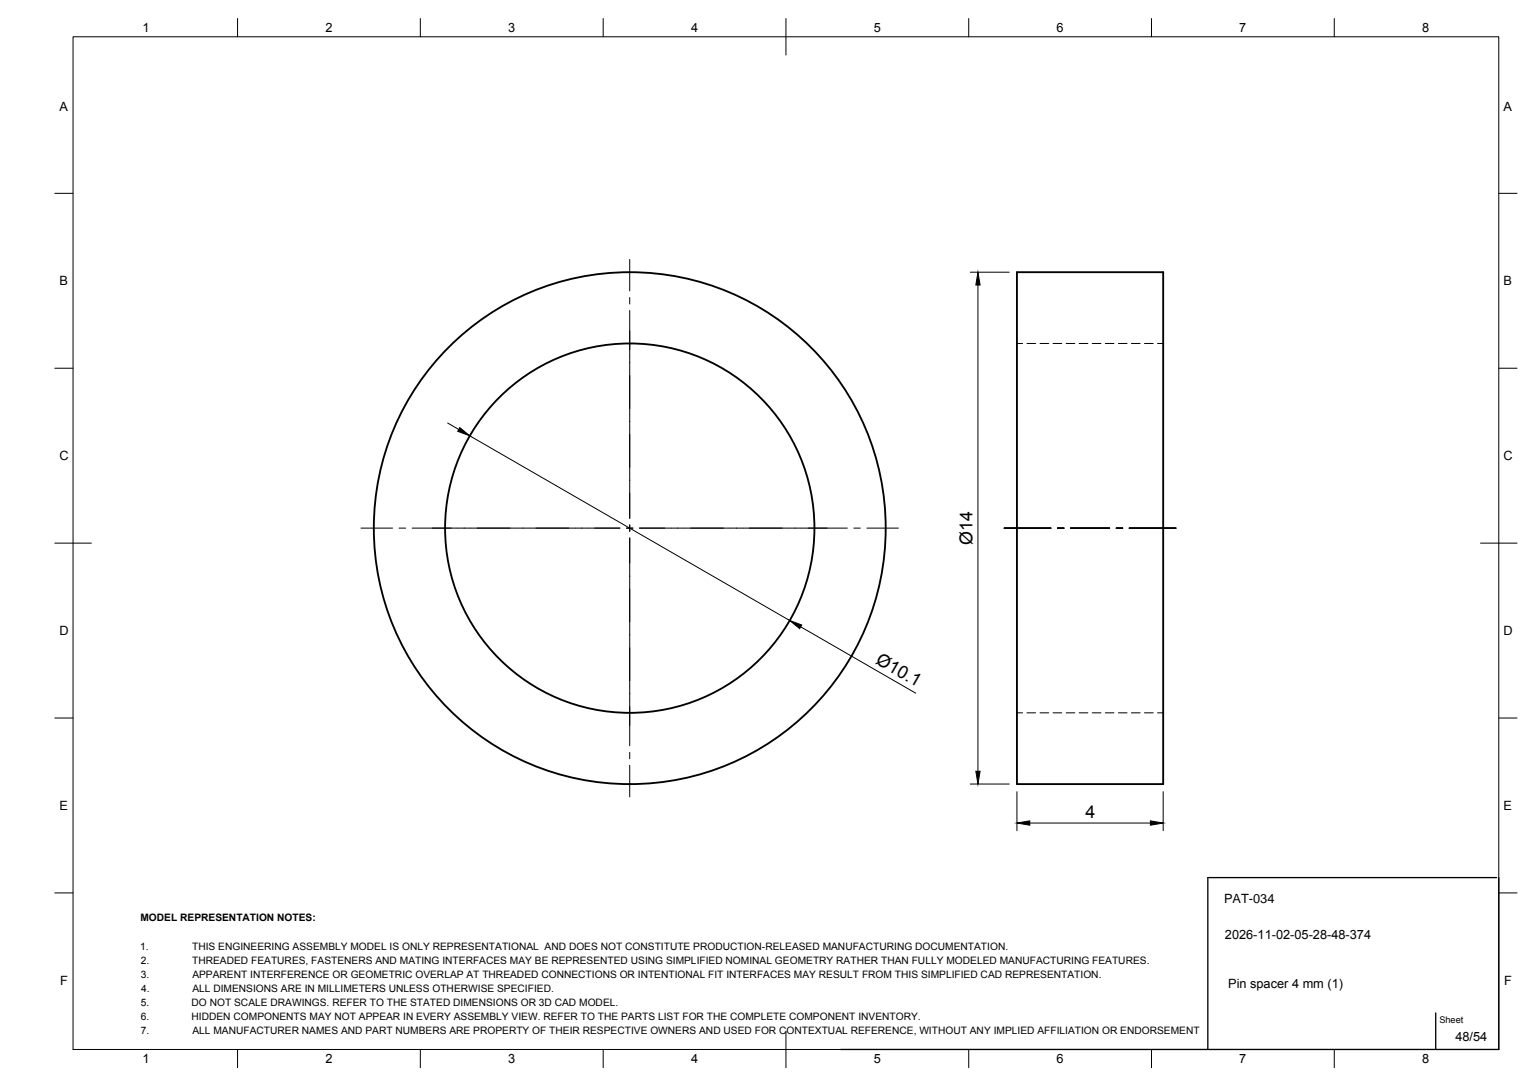
ISO-10303-21;
HEADER;
/* Generated by software containing ST-Developer
 * from STEP Tools, Inc. (www.steptools.com) 
 */

FILE_DESCRIPTION(
/* description */ ('Fatigue rig crank-slider'),
/* implementation_level */ '2;1');

FILE_NAME(
/* name */ 'Pin spacer 4 mm (1).step',
/* time_stamp */ '2026-10-28T03:24:50-07:00',
/* author */ (''),
/* organization */ (''),
/* preprocessor_version */ 'ST-DEVELOPER v20.2',
/* originating_system */ 'Autodesk Translation Framework v15.17.0.0',
/* authorisation */ '');

FILE_SCHEMA (('AUTOMOTIVE_DESIGN { 1 0 10303 214 3 1 1 }'));
ENDSEC;

DATA;
#10=MECHANICAL_DESIGN_GEOMETRIC_PRESENTATION_REPRESENTATION('',(#637),#16911);
#528=SHAPE_REPRESENTATION_RELATIONSHIP('SRR','None',#17172,#578);
#578=ADVANCED_BREP_SHAPE_REPRESENTATION('',(#694),#16901);
#637=STYLED_ITEM('',(#17487),#694);
#694=MANIFOLD_SOLID_BREP('Body1',#8930);
#884=FACE_BOUND('',#2346,.T.);
#885=FACE_BOUND('',#2348,.T.);
#1140=PLANE('',#10330);
#1141=PLANE('',#10331);
#1636=FACE_OUTER_BOUND('',#2343,.T.);
#1637=FACE_OUTER_BOUND('',#2344,.T.);
#1638=FACE_OUTER_BOUND('',#2345,.T.);
#1639=FACE_OUTER_BOUND('',#2347,.T.);
#2343=EDGE_LOOP('',(#7732,#7733,#7734,#7735));
#2344=EDGE_LOOP('',(#7736,#7737,#7738,#7739));
#2345=EDGE_LOOP('',(#7740));
#2346=EDGE_LOOP('',(#7741));
#2347=EDGE_LOOP('',(#7742));
#2348=EDGE_LOOP('',(#7743));
#2925=LINE('',#16224,#3571);
#2926=LINE('',#16230,#3572);
#3571=VECTOR('',#12697,0.505000000000001);
#3572=VECTOR('',#12704,0.699999999999999);
#4101=CIRCLE('',#10325,0.505000000000001);
#4102=CIRCLE('',#10326,0.505000000000001);
#4103=CIRCLE('',#10328,0.699999999999999);
#4104=CIRCLE('',#10329,0.699999999999999);
#4745=VERTEX_POINT('',#16221);
#4746=VERTEX_POINT('',#16223);
#4747=VERTEX_POINT('',#16227);
#4748=VERTEX_POINT('',#16229);
#5764=EDGE_CURVE('',#4745,#4745,#4101,.T.);
#5765=EDGE_CURVE('',#4745,#4746,#2925,.T.);
#5766=EDGE_CURVE('',#4746,#4746,#4102,.T.);
#5767=EDGE_CURVE('',#4747,#4747,#4103,.T.);
#5768=EDGE_CURVE('',#4747,#4748,#2926,.T.);
#5769=EDGE_CURVE('',#4748,#4748,#4104,.T.);
#7732=ORIENTED_EDGE('',*,*,#5764,.F.);
#7733=ORIENTED_EDGE('',*,*,#5765,.T.);
#7734=ORIENTED_EDGE('',*,*,#5766,.T.);
#7735=ORIENTED_EDGE('',*,*,#5765,.F.);
#7736=ORIENTED_EDGE('',*,*,#5767,.F.);
#7737=ORIENTED_EDGE('',*,*,#5768,.T.);
#7738=ORIENTED_EDGE('',*,*,#5769,.T.);
#7739=ORIENTED_EDGE('',*,*,#5768,.F.);
#7740=ORIENTED_EDGE('',*,*,#5767,.T.);
#7741=ORIENTED_EDGE('',*,*,#5764,.T.);
#7742=ORIENTED_EDGE('',*,*,#5769,.F.);
#7743=ORIENTED_EDGE('',*,*,#5766,.F.);
#8339=CYLINDRICAL_SURFACE('',#10324,0.505000000000001);
#8340=CYLINDRICAL_SURFACE('',#10327,0.699999999999999);
#8774=ADVANCED_FACE('',(#1636),#8339,.F.);
#8775=ADVANCED_FACE('',(#1637),#8340,.T.);
#8776=ADVANCED_FACE('',(#1638,#884),#1140,.T.);
#8777=ADVANCED_FACE('',(#1639,#885),#1141,.F.);
#8930=CLOSED_SHELL('',(#8774,#8775,#8776,#8777));
#10323=AXIS2_PLACEMENT_3D('',#16219,#12691,#12692);
#10324=AXIS2_PLACEMENT_3D('',#16220,#12693,#12694);
#10325=AXIS2_PLACEMENT_3D('',#16222,#12695,#12696);
#10326=AXIS2_PLACEMENT_3D('',#16225,#12698,#12699);
#10327=AXIS2_PLACEMENT_3D('',#16226,#12700,#12701);
#10328=AXIS2_PLACEMENT_3D('',#16228,#12702,#12703);
#10329=AXIS2_PLACEMENT_3D('',#16231,#12705,#12706);
#10330=AXIS2_PLACEMENT_3D('',#16232,#12707,#12708);
#10331=AXIS2_PLACEMENT_3D('',#16233,#12709,#12710);
#12691=DIRECTION('axis',(0.,0.,1.));
#12692=DIRECTION('refdir',(1.,0.,0.));
#12693=DIRECTION('center_axis',(0.,1.,0.));
#12694=DIRECTION('ref_axis',(1.,0.,0.));
#12695=DIRECTION('center_axis',(0.,-1.,0.));
#12696=DIRECTION('ref_axis',(1.,0.,0.));
#12697=DIRECTION('',(0.,-1.,0.));
#12698=DIRECTION('center_axis',(0.,-1.,0.));
#12699=DIRECTION('ref_axis',(1.,0.,0.));
#12700=DIRECTION('center_axis',(0.,1.,0.));
#12701=DIRECTION('ref_axis',(1.,0.,0.));
#12702=DIRECTION('center_axis',(0.,1.,0.));
#12703=DIRECTION('ref_axis',(1.,0.,0.));
#12704=DIRECTION('',(0.,-1.,0.));
#12705=DIRECTION('center_axis',(0.,1.,0.));
#12706=DIRECTION('ref_axis',(1.,0.,0.));
#12707=DIRECTION('center_axis',(0.,1.,0.));
#12708=DIRECTION('ref_axis',(1.,0.,0.));
#12709=DIRECTION('center_axis',(0.,1.,0.));
#12710=DIRECTION('ref_axis',(1.,0.,0.));
#16219=CARTESIAN_POINT('',(0.,0.,0.));
#16220=CARTESIAN_POINT('Origin',(11.,4.4,12.));
#16221=CARTESIAN_POINT('',(10.495,4.8,12.));
#16222=CARTESIAN_POINT('Origin',(11.,4.8,12.));
#16223=CARTESIAN_POINT('',(10.495,4.4,12.));
#16224=CARTESIAN_POINT('',(10.495,4.4,12.));
#16225=CARTESIAN_POINT('Origin',(11.,4.4,12.));
#16226=CARTESIAN_POINT('Origin',(11.,4.4,12.));
#16227=CARTESIAN_POINT('',(10.3,4.8,12.));
#16228=CARTESIAN_POINT('Origin',(11.,4.8,12.));
#16229=CARTESIAN_POINT('',(10.3,4.4,12.));
#16230=CARTESIAN_POINT('',(10.3,4.4,12.));
#16231=CARTESIAN_POINT('Origin',(11.,4.4,12.));
#16232=CARTESIAN_POINT('Origin',(11.,4.8,12.));
#16233=CARTESIAN_POINT('Origin',(11.,4.4,12.));
#16842=UNCERTAINTY_MEASURE_WITH_UNIT(LENGTH_MEASURE(0.001),#16912,
'DISTANCE_ACCURACY_VALUE',
'Maximum model space distance between geometric entities at asserted c
onnectivities');
#16852=UNCERTAINTY_MEASURE_WITH_UNIT(LENGTH_MEASURE(0.001),#16912,
'DISTANCE_ACCURACY_VALUE',
'Maximum model space distance between geometric entities at asserted c
onnectivities');
#16901=(
GEOMETRIC_REPRESENTATION_CONTEXT(3)
GLOBAL_UNCERTAINTY_ASSIGNED_CONTEXT((#16842))
GLOBAL_UNIT_ASSIGNED_CONTEXT((#16912,#16914,#16915))
REPRESENTATION_CONTEXT('','3D')
);
#16911=(
GEOMETRIC_REPRESENTATION_CONTEXT(3)
GLOBAL_UNCERTAINTY_ASSIGNED_CONTEXT((#16852))
GLOBAL_UNIT_ASSIGNED_CONTEXT((#16912,#16914,#16915))
REPRESENTATION_CONTEXT('','3D')
);
#16912=(
LENGTH_UNIT()
NAMED_UNIT(*)
SI_UNIT(.CENTI.,.METRE.)
);
#16914=(
NAMED_UNIT(*)
PLANE_ANGLE_UNIT()
SI_UNIT($,.RADIAN.)
);
#16915=(
NAMED_UNIT(*)
SI_UNIT($,.STERADIAN.)
SOLID_ANGLE_UNIT()
);
#16964=SHAPE_DEFINITION_REPRESENTATION(#17036,#17172);
#17036=PRODUCT_DEFINITION_SHAPE('',$,#17231);
#17172=SHAPE_REPRESENTATION('',(#10323),#16901);
#17182=PRODUCT_DEFINITION_CONTEXT('part definition',#17358,'design');
#17231=PRODUCT_DEFINITION('Pin spacer 4 mm (1)','Pin spacer 4 mm (1)',#17289,
#17182);
#17289=PRODUCT_DEFINITION_FORMATION('',$,#17408);
#17358=APPLICATION_CONTEXT(
'Core Data for Automotive Mechanical Design Process');
#17359=PRODUCT_CONTEXT('part definition',#17358,'mechanical');
#17408=PRODUCT('Pin spacer 4 mm (1)','Pin spacer 4 mm (1)',
'Pin spacer 4 mm (1)',(#17359));
#17481=COLOUR_RGB('Grey',0.48,0.52,0.57);
#17482=FILL_AREA_STYLE_COLOUR('',#17481);
#17483=FILL_AREA_STYLE('',(#17482));
#17484=SURFACE_STYLE_FILL_AREA(#17483);
#17485=SURFACE_SIDE_STYLE('',(#17484));
#17486=SURFACE_STYLE_USAGE(.BOTH.,#17485);
#17487=PRESENTATION_STYLE_ASSIGNMENT((#17486));
ENDSEC;
END-ISO-10303-21;
